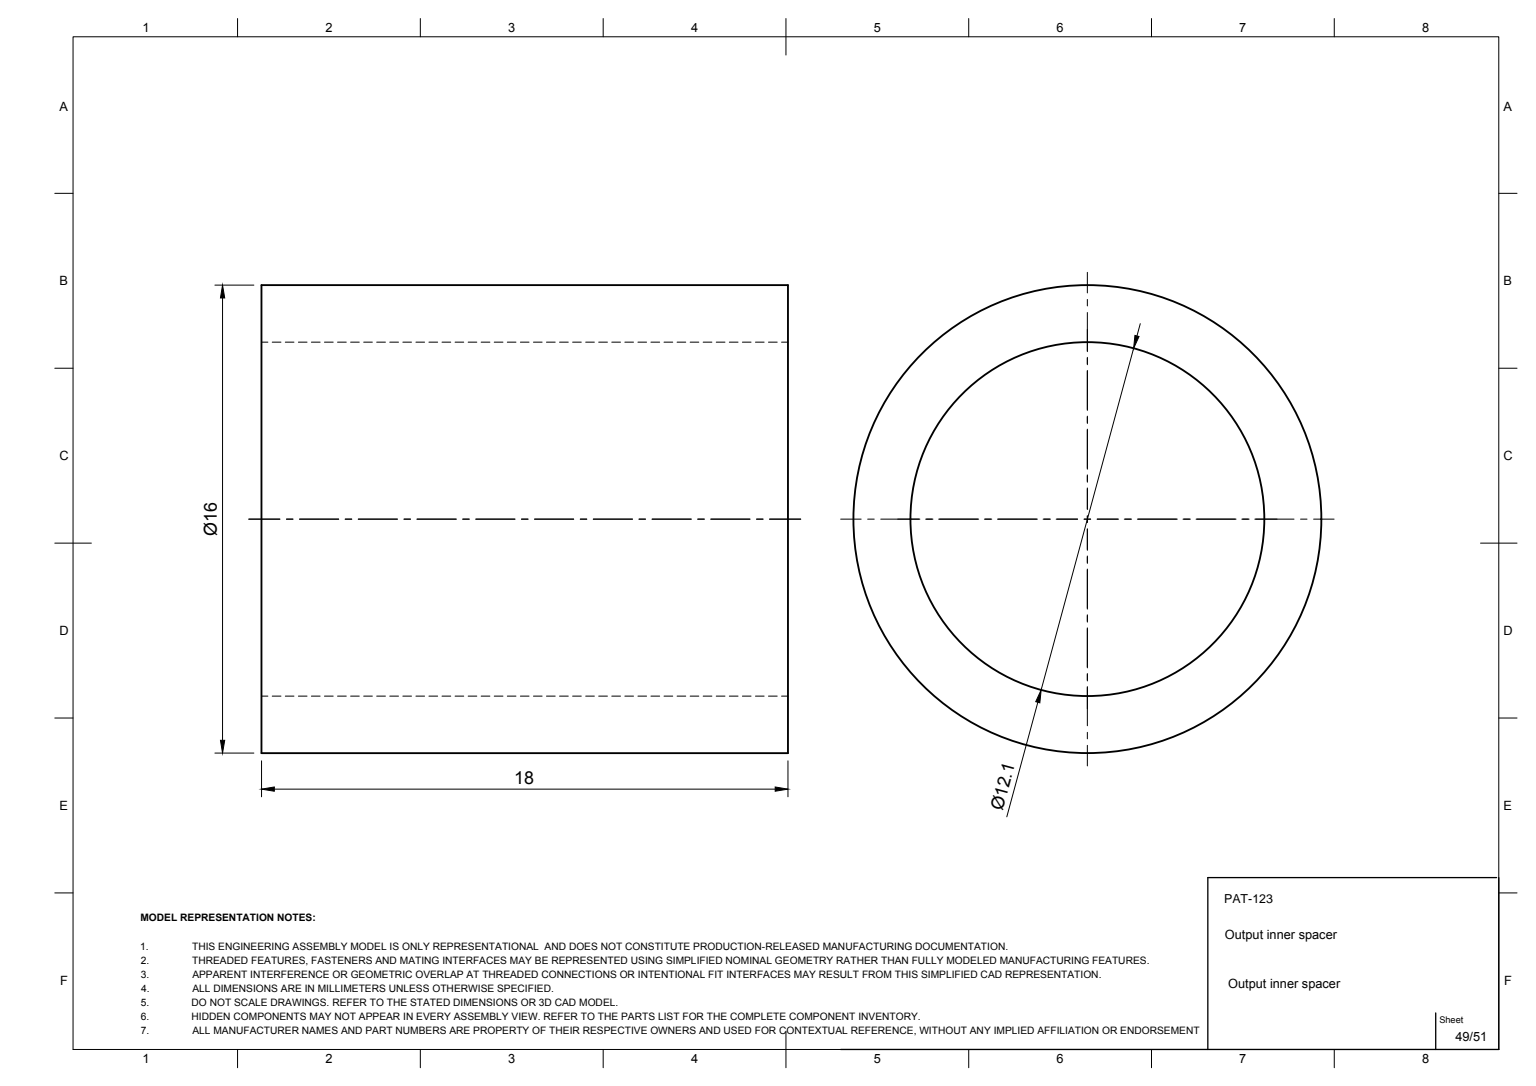
ISO-10303-21;
HEADER;
/* Generated by software containing ST-Developer
 * from STEP Tools, Inc. (www.steptools.com) 
 */

FILE_DESCRIPTION(
/* description */ ('Worm-less right-angle friction wheel drive'),
/* implementation_level */ '2;1');

FILE_NAME(
/* name */ 'Output inner spacer.step',
/* time_stamp */ '2026-10-28T03:22:36-07:00',
/* author */ (''),
/* organization */ (''),
/* preprocessor_version */ 'ST-DEVELOPER v20.2',
/* originating_system */ 'Autodesk Translation Framework v15.17.0.0',
/* authorisation */ '');

FILE_SCHEMA (('AUTOMOTIVE_DESIGN { 1 0 10303 214 3 1 1 }'));
ENDSEC;

DATA;
#10=MECHANICAL_DESIGN_GEOMETRIC_PRESENTATION_REPRESENTATION('',(#660),#17046);
#559=SHAPE_REPRESENTATION_RELATIONSHIP('SRR','None',#17305,#606);
#606=ADVANCED_BREP_SHAPE_REPRESENTATION('',(#710),#17041);
#660=STYLED_ITEM('',(#17584),#710);
#710=MANIFOLD_SOLID_BREP('Body1',#8219);
#945=FACE_BOUND('',#2334,.T.);
#946=FACE_BOUND('',#2336,.T.);
#1179=PLANE('',#9696);
#1180=PLANE('',#9697);
#1635=FACE_OUTER_BOUND('',#2331,.T.);
#1636=FACE_OUTER_BOUND('',#2332,.T.);
#1637=FACE_OUTER_BOUND('',#2333,.T.);
#1638=FACE_OUTER_BOUND('',#2335,.T.);
#2331=EDGE_LOOP('',(#7344,#7345,#7346,#7347));
#2332=EDGE_LOOP('',(#7348,#7349,#7350,#7351));
#2333=EDGE_LOOP('',(#7352));
#2334=EDGE_LOOP('',(#7353));
#2335=EDGE_LOOP('',(#7354));
#2336=EDGE_LOOP('',(#7355));
#2857=LINE('',#16617,#3397);
#2858=LINE('',#16623,#3398);
#3397=VECTOR('',#12153,0.605);
#3398=VECTOR('',#12160,0.8);
#3850=CIRCLE('',#9691,0.605);
#3851=CIRCLE('',#9692,0.605);
#3852=CIRCLE('',#9694,0.8);
#3853=CIRCLE('',#9695,0.8);
#4475=VERTEX_POINT('',#16614);
#4476=VERTEX_POINT('',#16616);
#4477=VERTEX_POINT('',#16620);
#4478=VERTEX_POINT('',#16622);
#5441=EDGE_CURVE('',#4475,#4475,#3850,.T.);
#5442=EDGE_CURVE('',#4475,#4476,#2857,.T.);
#5443=EDGE_CURVE('',#4476,#4476,#3851,.T.);
#5444=EDGE_CURVE('',#4477,#4477,#3852,.T.);
#5445=EDGE_CURVE('',#4477,#4478,#2858,.T.);
#5446=EDGE_CURVE('',#4478,#4478,#3853,.T.);
#7344=ORIENTED_EDGE('',*,*,#5441,.F.);
#7345=ORIENTED_EDGE('',*,*,#5442,.T.);
#7346=ORIENTED_EDGE('',*,*,#5443,.T.);
#7347=ORIENTED_EDGE('',*,*,#5442,.F.);
#7348=ORIENTED_EDGE('',*,*,#5444,.F.);
#7349=ORIENTED_EDGE('',*,*,#5445,.T.);
#7350=ORIENTED_EDGE('',*,*,#5446,.T.);
#7351=ORIENTED_EDGE('',*,*,#5445,.F.);
#7352=ORIENTED_EDGE('',*,*,#5444,.T.);
#7353=ORIENTED_EDGE('',*,*,#5441,.T.);
#7354=ORIENTED_EDGE('',*,*,#5446,.F.);
#7355=ORIENTED_EDGE('',*,*,#5443,.F.);
#7691=CYLINDRICAL_SURFACE('',#9690,0.605);
#7692=CYLINDRICAL_SURFACE('',#9693,0.8);
#8127=ADVANCED_FACE('',(#1635),#7691,.F.);
#8128=ADVANCED_FACE('',(#1636),#7692,.T.);
#8129=ADVANCED_FACE('',(#1637,#945),#1179,.T.);
#8130=ADVANCED_FACE('',(#1638,#946),#1180,.F.);
#8219=CLOSED_SHELL('',(#8127,#8128,#8129,#8130));
#9689=AXIS2_PLACEMENT_3D('',#16612,#12147,#12148);
#9690=AXIS2_PLACEMENT_3D('',#16613,#12149,#12150);
#9691=AXIS2_PLACEMENT_3D('',#16615,#12151,#12152);
#9692=AXIS2_PLACEMENT_3D('',#16618,#12154,#12155);
#9693=AXIS2_PLACEMENT_3D('',#16619,#12156,#12157);
#9694=AXIS2_PLACEMENT_3D('',#16621,#12158,#12159);
#9695=AXIS2_PLACEMENT_3D('',#16624,#12161,#12162);
#9696=AXIS2_PLACEMENT_3D('',#16625,#12163,#12164);
#9697=AXIS2_PLACEMENT_3D('',#16626,#12165,#12166);
#12147=DIRECTION('axis',(0.,0.,1.));
#12148=DIRECTION('refdir',(1.,0.,0.));
#12149=DIRECTION('center_axis',(1.,0.,0.));
#12150=DIRECTION('ref_axis',(0.,0.,-1.));
#12151=DIRECTION('center_axis',(-1.,0.,0.));
#12152=DIRECTION('ref_axis',(0.,0.,-1.));
#12153=DIRECTION('',(-1.,0.,0.));
#12154=DIRECTION('center_axis',(-1.,0.,0.));
#12155=DIRECTION('ref_axis',(0.,0.,-1.));
#12156=DIRECTION('center_axis',(1.,0.,0.));
#12157=DIRECTION('ref_axis',(0.,0.,-1.));
#12158=DIRECTION('center_axis',(1.,0.,0.));
#12159=DIRECTION('ref_axis',(0.,0.,-1.));
#12160=DIRECTION('',(-1.,0.,0.));
#12161=DIRECTION('center_axis',(1.,0.,0.));
#12162=DIRECTION('ref_axis',(0.,0.,-1.));
#12163=DIRECTION('center_axis',(1.,0.,0.));
#12164=DIRECTION('ref_axis',(0.,0.,-1.));
#12165=DIRECTION('center_axis',(1.,0.,0.));
#12166=DIRECTION('ref_axis',(0.,0.,-1.));
#16612=CARTESIAN_POINT('',(0.,0.,0.));
#16613=CARTESIAN_POINT('Origin',(3.2,3.,7.));
#16614=CARTESIAN_POINT('',(5.,3.,7.605));
#16615=CARTESIAN_POINT('Origin',(5.,3.,7.));
#16616=CARTESIAN_POINT('',(3.2,3.,7.605));
#16617=CARTESIAN_POINT('',(3.2,3.,7.605));
#16618=CARTESIAN_POINT('Origin',(3.2,3.,7.));
#16619=CARTESIAN_POINT('Origin',(3.2,3.,7.));
#16620=CARTESIAN_POINT('',(5.,3.,7.8));
#16621=CARTESIAN_POINT('Origin',(5.,3.,7.));
#16622=CARTESIAN_POINT('',(3.2,3.,7.8));
#16623=CARTESIAN_POINT('',(3.2,3.,7.8));
#16624=CARTESIAN_POINT('Origin',(3.2,3.,7.));
#16625=CARTESIAN_POINT('Origin',(5.,3.,7.));
#16626=CARTESIAN_POINT('Origin',(3.2,3.,7.));
#16988=UNCERTAINTY_MEASURE_WITH_UNIT(LENGTH_MEASURE(0.001),#17047,
'DISTANCE_ACCURACY_VALUE',
'Maximum model space distance between geometric entities at asserted c
onnectivities');
#16993=UNCERTAINTY_MEASURE_WITH_UNIT(LENGTH_MEASURE(0.001),#17047,
'DISTANCE_ACCURACY_VALUE',
'Maximum model space distance between geometric entities at asserted c
onnectivities');
#17041=(
GEOMETRIC_REPRESENTATION_CONTEXT(3)
GLOBAL_UNCERTAINTY_ASSIGNED_CONTEXT((#16988))
GLOBAL_UNIT_ASSIGNED_CONTEXT((#17047,#17049,#17050))
REPRESENTATION_CONTEXT('','3D')
);
#17046=(
GEOMETRIC_REPRESENTATION_CONTEXT(3)
GLOBAL_UNCERTAINTY_ASSIGNED_CONTEXT((#16993))
GLOBAL_UNIT_ASSIGNED_CONTEXT((#17047,#17049,#17050))
REPRESENTATION_CONTEXT('','3D')
);
#17047=(
LENGTH_UNIT()
NAMED_UNIT(*)
SI_UNIT(.CENTI.,.METRE.)
);
#17049=(
NAMED_UNIT(*)
PLANE_ANGLE_UNIT()
SI_UNIT($,.RADIAN.)
);
#17050=(
NAMED_UNIT(*)
SI_UNIT($,.STERADIAN.)
SOLID_ANGLE_UNIT()
);
#17098=SHAPE_DEFINITION_REPRESENTATION(#17232,#17305);
#17232=PRODUCT_DEFINITION_SHAPE('',$,#17358);
#17305=SHAPE_REPRESENTATION('',(#9689),#17041);
#17310=PRODUCT_DEFINITION_CONTEXT('part definition',#17468,'design');
#17358=PRODUCT_DEFINITION('Output inner spacer','Output inner spacer',#17410,
#17310);
#17410=PRODUCT_DEFINITION_FORMATION('',$,#17517);
#17468=APPLICATION_CONTEXT(
'Core Data for Automotive Mechanical Design Process');
#17469=PRODUCT_CONTEXT('part definition',#17468,'mechanical');
#17517=PRODUCT('Output inner spacer','Output inner spacer',
'Output inner spacer',(#17469));
#17578=COLOUR_RGB('Sky Blue',0.24,0.69,0.87);
#17579=FILL_AREA_STYLE_COLOUR('',#17578);
#17580=FILL_AREA_STYLE('',(#17579));
#17581=SURFACE_STYLE_FILL_AREA(#17580);
#17582=SURFACE_SIDE_STYLE('',(#17581));
#17583=SURFACE_STYLE_USAGE(.BOTH.,#17582);
#17584=PRESENTATION_STYLE_ASSIGNMENT((#17583));
ENDSEC;
END-ISO-10303-21;
